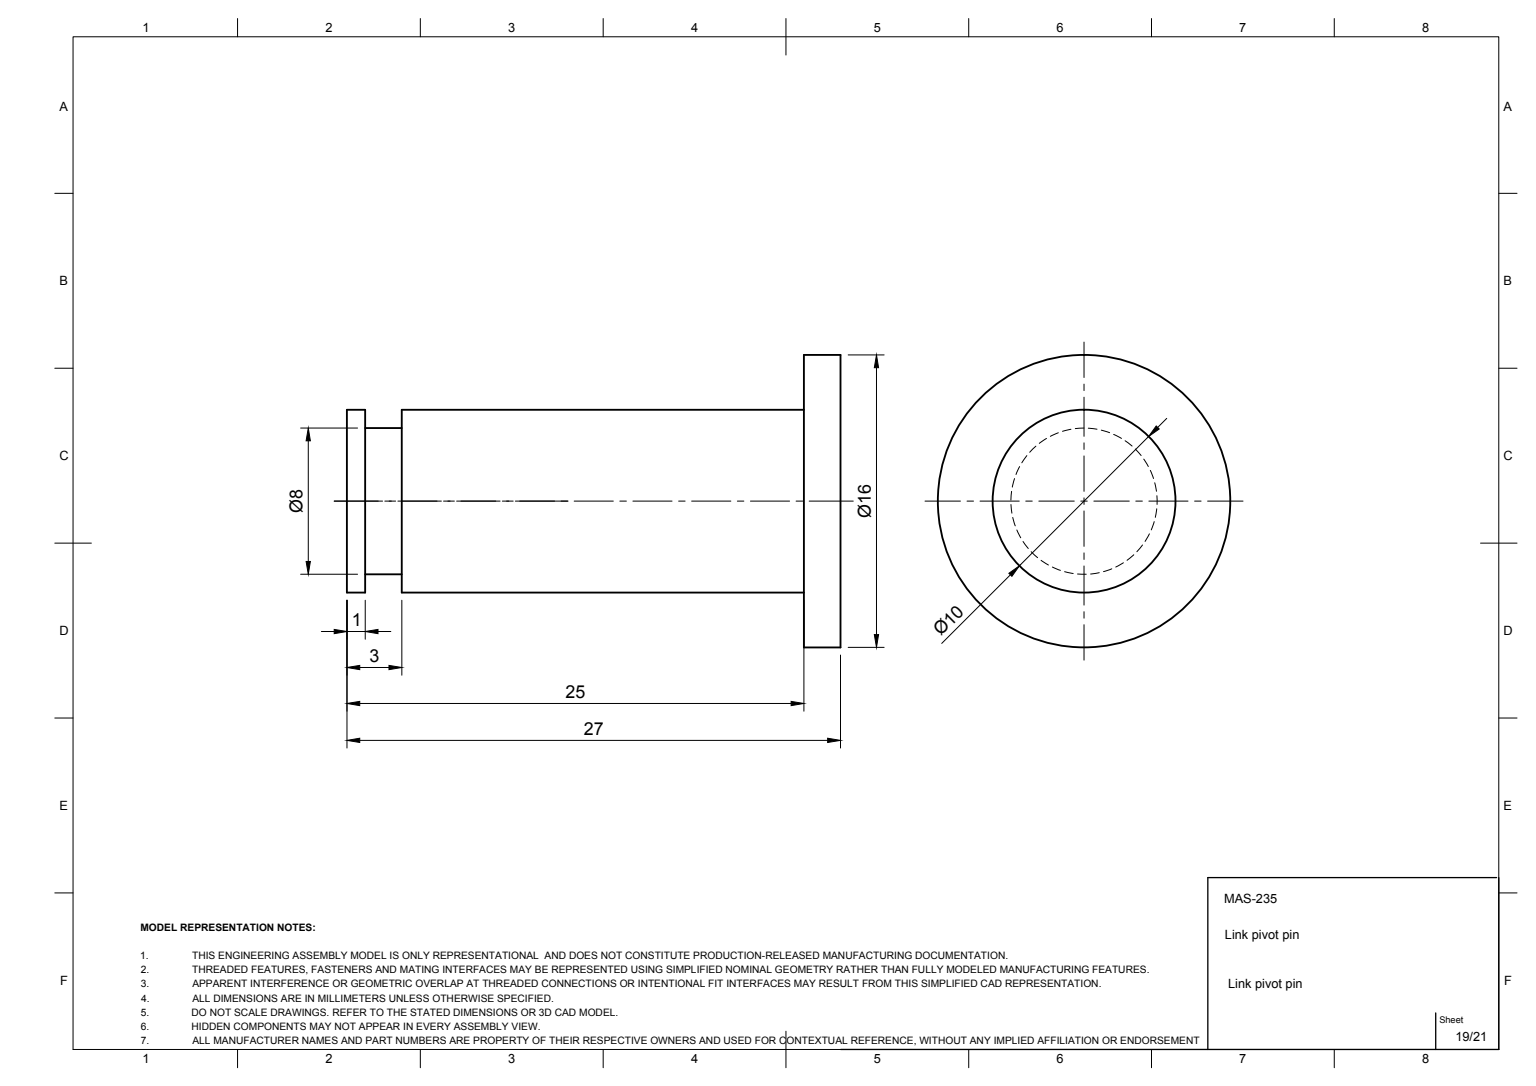
ISO-10303-21;
HEADER;
/* Generated by software containing ST-Developer
 * from STEP Tools, Inc. (www.steptools.com) 
 */

FILE_DESCRIPTION(
/* description */ ('Independent Whitworth quick-return mechanism. Crank radius40, ground-
center spacing80, lever180, connecting rod160, output guide X200. Nomi
nal stroke180 and long/short phase ratio2. Retained guide rods, replac
eable bearing sleeves and captured sliding shoe. No load or production
 rating assigned.'),
/* implementation_level */ '2;1');

FILE_NAME(
/* name */ 'Link pivot pin.step',
/* time_stamp */ '2026-11-09T18:22:56-08:00',
/* author */ (''),
/* organization */ (''),
/* preprocessor_version */ 'ST-DEVELOPER v20.2',
/* originating_system */ 'Autodesk Translation Framework v15.17.0.0',
/* authorisation */ '');

FILE_SCHEMA (('AUTOMOTIVE_DESIGN { 1 0 10303 214 3 1 1 }'));
ENDSEC;

DATA;
#10=MECHANICAL_DESIGN_GEOMETRIC_PRESENTATION_REPRESENTATION('',(#233),#4388);
#193=SHAPE_REPRESENTATION_RELATIONSHIP('SRR','None',#4492,#213);
#213=ADVANCED_BREP_SHAPE_REPRESENTATION('',(#253),#4382);
#233=STYLED_ITEM('',(#4595),#253);
#253=MANIFOLD_SOLID_BREP('Body1',#2338);
#307=FACE_BOUND('',#713,.T.);
#308=FACE_BOUND('',#715,.T.);
#309=FACE_BOUND('',#718,.T.);
#385=PLANE('',#2785);
#386=PLANE('',#2787);
#387=PLANE('',#2791);
#388=PLANE('',#2796);
#389=PLANE('',#2798);
#516=FACE_OUTER_BOUND('',#711,.T.);
#517=FACE_OUTER_BOUND('',#712,.T.);
#518=FACE_OUTER_BOUND('',#714,.T.);
#519=FACE_OUTER_BOUND('',#716,.T.);
#520=FACE_OUTER_BOUND('',#717,.T.);
#521=FACE_OUTER_BOUND('',#719,.T.);
#522=FACE_OUTER_BOUND('',#720,.T.);
#523=FACE_OUTER_BOUND('',#721,.T.);
#524=FACE_OUTER_BOUND('',#722,.T.);
#711=EDGE_LOOP('',(#2008,#2009,#2010,#2011));
#712=EDGE_LOOP('',(#2012));
#713=EDGE_LOOP('',(#2013));
#714=EDGE_LOOP('',(#2014));
#715=EDGE_LOOP('',(#2015));
#716=EDGE_LOOP('',(#2016,#2017,#2018,#2019));
#717=EDGE_LOOP('',(#2020));
#718=EDGE_LOOP('',(#2021));
#719=EDGE_LOOP('',(#2022,#2023,#2024,#2025));
#720=EDGE_LOOP('',(#2026));
#721=EDGE_LOOP('',(#2027,#2028,#2029,#2030));
#722=EDGE_LOOP('',(#2031));
#876=LINE('',#4176,#1015);
#877=LINE('',#4187,#1016);
#878=LINE('',#4195,#1017);
#879=LINE('',#4199,#1018);
#1015=VECTOR('',#3452,4.);
#1016=VECTOR('',#3467,5.);
#1017=VECTOR('',#3476,8.);
#1018=VECTOR('',#3483,5.);
#1127=CIRCLE('',#2783,4.);
#1128=CIRCLE('',#2784,4.);
#1129=CIRCLE('',#2786,5.);
#1130=CIRCLE('',#2788,5.);
#1131=CIRCLE('',#2790,5.);
#1132=CIRCLE('',#2792,8.);
#1133=CIRCLE('',#2793,5.);
#1134=CIRCLE('',#2795,8.);
#1297=VERTEX_POINT('',#4173);
#1298=VERTEX_POINT('',#4175);
#1299=VERTEX_POINT('',#4179);
#1300=VERTEX_POINT('',#4182);
#1301=VERTEX_POINT('',#4185);
#1302=VERTEX_POINT('',#4189);
#1303=VERTEX_POINT('',#4191);
#1304=VERTEX_POINT('',#4194);
#1540=EDGE_CURVE('',#1297,#1297,#1127,.T.);
#1541=EDGE_CURVE('',#1297,#1298,#876,.T.);
#1542=EDGE_CURVE('',#1298,#1298,#1128,.T.);
#1543=EDGE_CURVE('',#1299,#1299,#1129,.T.);
#1544=EDGE_CURVE('',#1300,#1300,#1130,.T.);
#1545=EDGE_CURVE('',#1301,#1301,#1131,.T.);
#1546=EDGE_CURVE('',#1301,#1300,#877,.T.);
#1547=EDGE_CURVE('',#1302,#1302,#1132,.T.);
#1548=EDGE_CURVE('',#1303,#1303,#1133,.T.);
#1549=EDGE_CURVE('',#1302,#1304,#878,.T.);
#1550=EDGE_CURVE('',#1304,#1304,#1134,.T.);
#1551=EDGE_CURVE('',#1299,#1303,#879,.T.);
#2008=ORIENTED_EDGE('',*,*,#1540,.T.);
#2009=ORIENTED_EDGE('',*,*,#1541,.T.);
#2010=ORIENTED_EDGE('',*,*,#1542,.F.);
#2011=ORIENTED_EDGE('',*,*,#1541,.F.);
#2012=ORIENTED_EDGE('',*,*,#1543,.F.);
#2013=ORIENTED_EDGE('',*,*,#1540,.F.);
#2014=ORIENTED_EDGE('',*,*,#1544,.F.);
#2015=ORIENTED_EDGE('',*,*,#1542,.T.);
#2016=ORIENTED_EDGE('',*,*,#1545,.F.);
#2017=ORIENTED_EDGE('',*,*,#1546,.T.);
#2018=ORIENTED_EDGE('',*,*,#1544,.T.);
#2019=ORIENTED_EDGE('',*,*,#1546,.F.);
#2020=ORIENTED_EDGE('',*,*,#1547,.T.);
#2021=ORIENTED_EDGE('',*,*,#1548,.F.);
#2022=ORIENTED_EDGE('',*,*,#1547,.F.);
#2023=ORIENTED_EDGE('',*,*,#1549,.T.);
#2024=ORIENTED_EDGE('',*,*,#1550,.T.);
#2025=ORIENTED_EDGE('',*,*,#1549,.F.);
#2026=ORIENTED_EDGE('',*,*,#1550,.F.);
#2027=ORIENTED_EDGE('',*,*,#1543,.T.);
#2028=ORIENTED_EDGE('',*,*,#1551,.T.);
#2029=ORIENTED_EDGE('',*,*,#1548,.T.);
#2030=ORIENTED_EDGE('',*,*,#1551,.F.);
#2031=ORIENTED_EDGE('',*,*,#1545,.T.);
#2161=CYLINDRICAL_SURFACE('',#2782,4.);
#2162=CYLINDRICAL_SURFACE('',#2789,5.);
#2163=CYLINDRICAL_SURFACE('',#2794,8.);
#2164=CYLINDRICAL_SURFACE('',#2797,5.);
#2288=ADVANCED_FACE('',(#516),#2161,.T.);
#2289=ADVANCED_FACE('',(#517,#307),#385,.F.);
#2290=ADVANCED_FACE('',(#518,#308),#386,.F.);
#2291=ADVANCED_FACE('',(#519),#2162,.T.);
#2292=ADVANCED_FACE('',(#520,#309),#387,.T.);
#2293=ADVANCED_FACE('',(#521),#2163,.T.);
#2294=ADVANCED_FACE('',(#522),#388,.F.);
#2295=ADVANCED_FACE('',(#523),#2164,.T.);
#2296=ADVANCED_FACE('',(#524),#389,.T.);
#2338=CLOSED_SHELL('',(#2288,#2289,#2290,#2291,#2292,#2293,#2294,#2295,
#2296));
#2781=AXIS2_PLACEMENT_3D('',#4171,#3446,#3447);
#2782=AXIS2_PLACEMENT_3D('',#4172,#3448,#3449);
#2783=AXIS2_PLACEMENT_3D('',#4174,#3450,#3451);
#2784=AXIS2_PLACEMENT_3D('',#4177,#3453,#3454);
#2785=AXIS2_PLACEMENT_3D('',#4178,#3455,#3456);
#2786=AXIS2_PLACEMENT_3D('',#4180,#3457,#3458);
#2787=AXIS2_PLACEMENT_3D('',#4181,#3459,#3460);
#2788=AXIS2_PLACEMENT_3D('',#4183,#3461,#3462);
#2789=AXIS2_PLACEMENT_3D('',#4184,#3463,#3464);
#2790=AXIS2_PLACEMENT_3D('',#4186,#3465,#3466);
#2791=AXIS2_PLACEMENT_3D('',#4188,#3468,#3469);
#2792=AXIS2_PLACEMENT_3D('',#4190,#3470,#3471);
#2793=AXIS2_PLACEMENT_3D('',#4192,#3472,#3473);
#2794=AXIS2_PLACEMENT_3D('',#4193,#3474,#3475);
#2795=AXIS2_PLACEMENT_3D('',#4196,#3477,#3478);
#2796=AXIS2_PLACEMENT_3D('',#4197,#3479,#3480);
#2797=AXIS2_PLACEMENT_3D('',#4198,#3481,#3482);
#2798=AXIS2_PLACEMENT_3D('',#4200,#3484,#3485);
#3446=DIRECTION('axis',(0.,0.,1.));
#3447=DIRECTION('refdir',(1.,0.,0.));
#3448=DIRECTION('center_axis',(0.,0.,1.));
#3449=DIRECTION('ref_axis',(1.,0.,0.));
#3450=DIRECTION('center_axis',(0.,0.,1.));
#3451=DIRECTION('ref_axis',(1.,0.,0.));
#3452=DIRECTION('',(0.,0.,1.));
#3453=DIRECTION('center_axis',(0.,0.,1.));
#3454=DIRECTION('ref_axis',(1.,0.,0.));
#3455=DIRECTION('center_axis',(0.,0.,-1.));
#3456=DIRECTION('ref_axis',(-1.,0.,0.));
#3457=DIRECTION('center_axis',(0.,0.,-1.));
#3458=DIRECTION('ref_axis',(1.,0.,0.));
#3459=DIRECTION('center_axis',(0.,0.,1.));
#3460=DIRECTION('ref_axis',(1.,0.,0.));
#3461=DIRECTION('center_axis',(0.,0.,1.));
#3462=DIRECTION('ref_axis',(1.,0.,0.));
#3463=DIRECTION('center_axis',(0.,0.,1.));
#3464=DIRECTION('ref_axis',(1.,0.,0.));
#3465=DIRECTION('center_axis',(0.,0.,1.));
#3466=DIRECTION('ref_axis',(1.,0.,0.));
#3467=DIRECTION('',(0.,0.,-1.));
#3468=DIRECTION('center_axis',(0.,0.,1.));
#3469=DIRECTION('ref_axis',(1.,0.,0.));
#3470=DIRECTION('center_axis',(0.,0.,1.));
#3471=DIRECTION('ref_axis',(1.,0.,0.));
#3472=DIRECTION('center_axis',(0.,0.,1.));
#3473=DIRECTION('ref_axis',(1.,0.,0.));
#3474=DIRECTION('center_axis',(0.,0.,1.));
#3475=DIRECTION('ref_axis',(1.,0.,0.));
#3476=DIRECTION('',(0.,0.,-1.));
#3477=DIRECTION('center_axis',(0.,0.,1.));
#3478=DIRECTION('ref_axis',(1.,0.,0.));
#3479=DIRECTION('center_axis',(0.,0.,1.));
#3480=DIRECTION('ref_axis',(1.,0.,0.));
#3481=DIRECTION('center_axis',(0.,0.,1.));
#3482=DIRECTION('ref_axis',(1.,0.,0.));
#3483=DIRECTION('',(0.,0.,-1.));
#3484=DIRECTION('center_axis',(0.,0.,1.));
#3485=DIRECTION('ref_axis',(1.,0.,0.));
#4171=CARTESIAN_POINT('',(0.,0.,0.));
#4172=CARTESIAN_POINT('Origin',(0.,0.,23.));
#4173=CARTESIAN_POINT('',(-4.,-4.89858719658941E-16,22.));
#4174=CARTESIAN_POINT('Origin',(0.,0.,22.));
#4175=CARTESIAN_POINT('',(-4.,-4.89858719658941E-16,24.));
#4176=CARTESIAN_POINT('',(-4.,-4.89858719658941E-16,23.));
#4177=CARTESIAN_POINT('Origin',(0.,0.,24.));
#4178=CARTESIAN_POINT('Origin',(8.,0.,22.));
#4179=CARTESIAN_POINT('',(-5.,6.12323399573677E-16,22.));
#4180=CARTESIAN_POINT('Origin',(0.,0.,22.));
#4181=CARTESIAN_POINT('Origin',(4.,0.,24.));
#4182=CARTESIAN_POINT('',(-5.,-6.12323399573677E-16,24.));
#4183=CARTESIAN_POINT('Origin',(0.,0.,24.));
#4184=CARTESIAN_POINT('Origin',(0.,0.,0.));
#4185=CARTESIAN_POINT('',(-5.,-6.12323399573677E-16,25.));
#4186=CARTESIAN_POINT('Origin',(0.,0.,25.));
#4187=CARTESIAN_POINT('',(-5.,-6.12323399573677E-16,0.));
#4188=CARTESIAN_POINT('Origin',(0.,0.,0.));
#4189=CARTESIAN_POINT('',(-8.,-9.79717439317883E-16,0.));
#4190=CARTESIAN_POINT('Origin',(0.,0.,0.));
#4191=CARTESIAN_POINT('',(-5.,-6.12323399573677E-16,0.));
#4192=CARTESIAN_POINT('Origin',(0.,0.,0.));
#4193=CARTESIAN_POINT('Origin',(0.,0.,-2.));
#4194=CARTESIAN_POINT('',(-8.,-9.79717439317883E-16,-2.));
#4195=CARTESIAN_POINT('',(-8.,-9.79717439317883E-16,-2.));
#4196=CARTESIAN_POINT('Origin',(0.,0.,-2.));
#4197=CARTESIAN_POINT('Origin',(0.,0.,-2.));
#4198=CARTESIAN_POINT('Origin',(0.,0.,0.));
#4199=CARTESIAN_POINT('',(-5.,-6.12323399573677E-16,0.));
#4200=CARTESIAN_POINT('Origin',(0.,0.,25.));
#4360=UNCERTAINTY_MEASURE_WITH_UNIT(LENGTH_MEASURE(0.01),#4389,
'DISTANCE_ACCURACY_VALUE',
'Maximum model space distance between geometric entities at asserted c
onnectivities');
#4366=UNCERTAINTY_MEASURE_WITH_UNIT(LENGTH_MEASURE(0.01),#4389,
'DISTANCE_ACCURACY_VALUE',
'Maximum model space distance between geometric entities at asserted c
onnectivities');
#4382=(
GEOMETRIC_REPRESENTATION_CONTEXT(3)
GLOBAL_UNCERTAINTY_ASSIGNED_CONTEXT((#4360))
GLOBAL_UNIT_ASSIGNED_CONTEXT((#4389,#4391,#4392))
REPRESENTATION_CONTEXT('','3D')
);
#4388=(
GEOMETRIC_REPRESENTATION_CONTEXT(3)
GLOBAL_UNCERTAINTY_ASSIGNED_CONTEXT((#4366))
GLOBAL_UNIT_ASSIGNED_CONTEXT((#4389,#4391,#4392))
REPRESENTATION_CONTEXT('','3D')
);
#4389=(
LENGTH_UNIT()
NAMED_UNIT(*)
SI_UNIT(.MILLI.,.METRE.)
);
#4391=(
NAMED_UNIT(*)
PLANE_ANGLE_UNIT()
SI_UNIT($,.RADIAN.)
);
#4392=(
NAMED_UNIT(*)
SI_UNIT($,.STERADIAN.)
SOLID_ANGLE_UNIT()
);
#4408=SHAPE_DEFINITION_REPRESENTATION(#4429,#4492);
#4429=PRODUCT_DEFINITION_SHAPE('',$,#4514);
#4492=SHAPE_REPRESENTATION('',(#2781),#4382);
#4498=PRODUCT_DEFINITION_CONTEXT('part definition',#4563,'design');
#4514=PRODUCT_DEFINITION('Link pivot pin','Link pivot pin',#4535,#4498);
#4535=PRODUCT_DEFINITION_FORMATION('',$,#4580);
#4563=APPLICATION_CONTEXT(
'Core Data for Automotive Mechanical Design Process');
#4564=PRODUCT_CONTEXT('part definition',#4563,'mechanical');
#4580=PRODUCT('Link pivot pin','Link pivot pin',$,(#4564));
#4595=PRESENTATION_STYLE_ASSIGNMENT((#4609));
#4609=SURFACE_STYLE_USAGE(.BOTH.,#4623);
#4623=SURFACE_SIDE_STYLE('',(#4637));
#4637=SURFACE_STYLE_FILL_AREA(#4651);
#4651=FILL_AREA_STYLE('Pivot gray',(#4665));
#4665=FILL_AREA_STYLE_COLOUR('Pivot gray',#4679);
#4679=COLOUR_RGB('Pivot gray',0.407843137254902,0.447058823529412,0.498039215686275);
ENDSEC;
END-ISO-10303-21;
